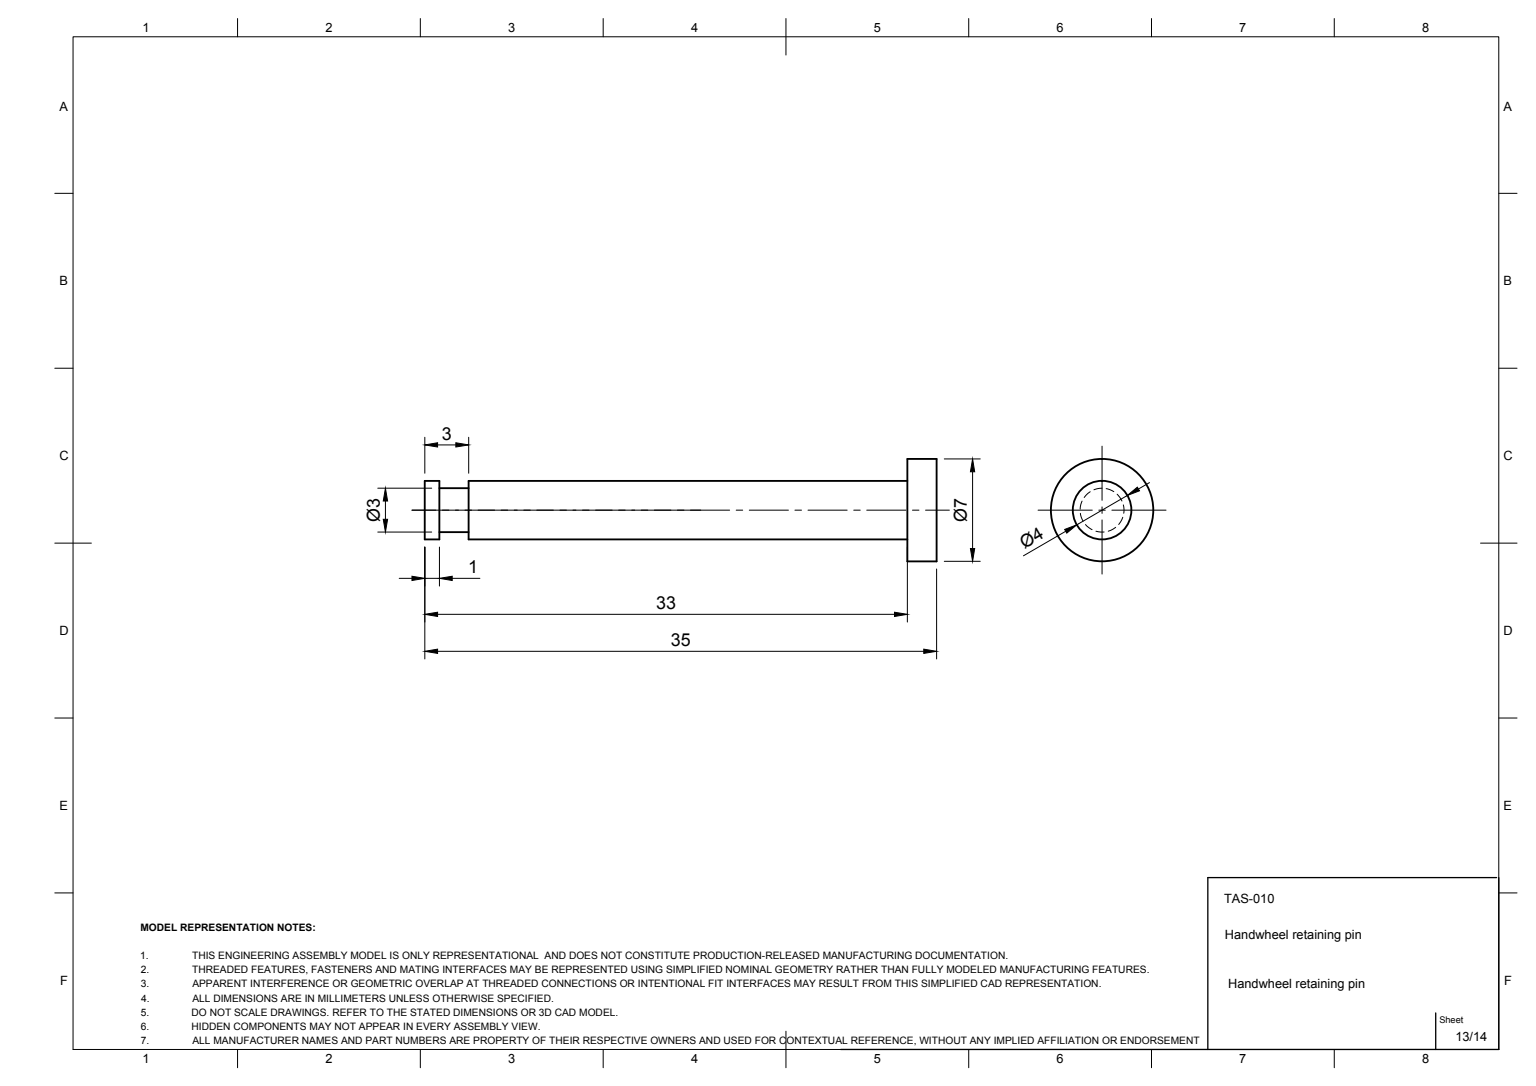
ISO-10303-21;
HEADER;
/* Generated by software containing ST-Developer
 * from STEP Tools, Inc. (www.steptools.com) 
 */

FILE_DESCRIPTION(
/* description */ (
'Independent keyed-quill tailstock, native coupled50mm slider andM16x2
 feed screw, conical dead center, bronze sleeves/thrust washers, cross
-pinned handwheel and bolted guide key. Custom center taper; no standa
rd taper compatibility, machine-bed compatibility or load rating assig
ned.'),
/* implementation_level */ '2;1');

FILE_NAME(
/* name */ 'Handwheel retaining pin.step',
/* time_stamp */ '2026-11-14T07:17:36-08:00',
/* author */ (''),
/* organization */ (''),
/* preprocessor_version */ 'ST-DEVELOPER v20.2',
/* originating_system */ 'Autodesk Translation Framework v15.17.0.0',
/* authorisation */ '');

FILE_SCHEMA (('AUTOMOTIVE_DESIGN { 1 0 10303 214 3 1 1 }'));
ENDSEC;

DATA;
#10=MECHANICAL_DESIGN_GEOMETRIC_PRESENTATION_REPRESENTATION('',(#163),#289387);
#129=SHAPE_REPRESENTATION_RELATIONSHIP('SRR','None',#289464,#146);
#146=ADVANCED_BREP_SHAPE_REPRESENTATION('',(#180),#289380);
#163=STYLED_ITEM('',(#289548),#180);
#180=MANIFOLD_SOLID_BREP('Body1',#16851);
#260=FACE_BOUND('',#1681,.T.);
#261=FACE_BOUND('',#1683,.T.);
#262=FACE_BOUND('',#1686,.T.);
#380=PLANE('',#17704);
#381=PLANE('',#17706);
#382=PLANE('',#17710);
#383=PLANE('',#17715);
#384=PLANE('',#17717);
#956=FACE_OUTER_BOUND('',#1679,.T.);
#957=FACE_OUTER_BOUND('',#1680,.T.);
#958=FACE_OUTER_BOUND('',#1682,.T.);
#959=FACE_OUTER_BOUND('',#1684,.T.);
#960=FACE_OUTER_BOUND('',#1685,.T.);
#961=FACE_OUTER_BOUND('',#1687,.T.);
#962=FACE_OUTER_BOUND('',#1688,.T.);
#963=FACE_OUTER_BOUND('',#1689,.T.);
#964=FACE_OUTER_BOUND('',#1690,.T.);
#1679=EDGE_LOOP('',(#14773,#14774,#14775,#14776));
#1680=EDGE_LOOP('',(#14777));
#1681=EDGE_LOOP('',(#14778));
#1682=EDGE_LOOP('',(#14779));
#1683=EDGE_LOOP('',(#14780));
#1684=EDGE_LOOP('',(#14781,#14782,#14783,#14784));
#1685=EDGE_LOOP('',(#14785));
#1686=EDGE_LOOP('',(#14786));
#1687=EDGE_LOOP('',(#14787,#14788,#14789,#14790));
#1688=EDGE_LOOP('',(#14791));
#1689=EDGE_LOOP('',(#14792,#14793,#14794,#14795));
#1690=EDGE_LOOP('',(#14796));
#1943=CIRCLE('',#17702,1.5);
#1944=CIRCLE('',#17703,1.5);
#1945=CIRCLE('',#17705,2.);
#1946=CIRCLE('',#17707,2.);
#1947=CIRCLE('',#17709,2.);
#1948=CIRCLE('',#17711,3.5);
#1949=CIRCLE('',#17712,2.);
#1950=CIRCLE('',#17714,3.5);
#4456=LINE('',#247266,#5093);
#4457=LINE('',#247277,#5094);
#4458=LINE('',#247285,#5095);
#4459=LINE('',#247289,#5096);
#5093=VECTOR('',#19718,1.5);
#5094=VECTOR('',#19733,2.);
#5095=VECTOR('',#19742,3.5);
#5096=VECTOR('',#19749,2.);
#7023=VERTEX_POINT('',#247263);
#7024=VERTEX_POINT('',#247265);
#7025=VERTEX_POINT('',#247269);
#7026=VERTEX_POINT('',#247272);
#7027=VERTEX_POINT('',#247275);
#7028=VERTEX_POINT('',#247279);
#7029=VERTEX_POINT('',#247281);
#7030=VERTEX_POINT('',#247284);
#9698=EDGE_CURVE('',#7023,#7023,#1943,.T.);
#9699=EDGE_CURVE('',#7023,#7024,#4456,.T.);
#9700=EDGE_CURVE('',#7024,#7024,#1944,.T.);
#9701=EDGE_CURVE('',#7025,#7025,#1945,.T.);
#9702=EDGE_CURVE('',#7026,#7026,#1946,.T.);
#9703=EDGE_CURVE('',#7027,#7027,#1947,.T.);
#9704=EDGE_CURVE('',#7027,#7026,#4457,.T.);
#9705=EDGE_CURVE('',#7028,#7028,#1948,.T.);
#9706=EDGE_CURVE('',#7029,#7029,#1949,.T.);
#9707=EDGE_CURVE('',#7028,#7030,#4458,.T.);
#9708=EDGE_CURVE('',#7030,#7030,#1950,.T.);
#9709=EDGE_CURVE('',#7025,#7029,#4459,.T.);
#14773=ORIENTED_EDGE('',*,*,#9698,.F.);
#14774=ORIENTED_EDGE('',*,*,#9699,.T.);
#14775=ORIENTED_EDGE('',*,*,#9700,.T.);
#14776=ORIENTED_EDGE('',*,*,#9699,.F.);
#14777=ORIENTED_EDGE('',*,*,#9701,.F.);
#14778=ORIENTED_EDGE('',*,*,#9700,.F.);
#14779=ORIENTED_EDGE('',*,*,#9702,.F.);
#14780=ORIENTED_EDGE('',*,*,#9698,.T.);
#14781=ORIENTED_EDGE('',*,*,#9703,.F.);
#14782=ORIENTED_EDGE('',*,*,#9704,.T.);
#14783=ORIENTED_EDGE('',*,*,#9702,.T.);
#14784=ORIENTED_EDGE('',*,*,#9704,.F.);
#14785=ORIENTED_EDGE('',*,*,#9705,.T.);
#14786=ORIENTED_EDGE('',*,*,#9706,.F.);
#14787=ORIENTED_EDGE('',*,*,#9705,.F.);
#14788=ORIENTED_EDGE('',*,*,#9707,.T.);
#14789=ORIENTED_EDGE('',*,*,#9708,.T.);
#14790=ORIENTED_EDGE('',*,*,#9707,.F.);
#14791=ORIENTED_EDGE('',*,*,#9708,.F.);
#14792=ORIENTED_EDGE('',*,*,#9701,.T.);
#14793=ORIENTED_EDGE('',*,*,#9709,.T.);
#14794=ORIENTED_EDGE('',*,*,#9706,.T.);
#14795=ORIENTED_EDGE('',*,*,#9709,.F.);
#14796=ORIENTED_EDGE('',*,*,#9703,.T.);
#16128=CYLINDRICAL_SURFACE('',#17701,1.5);
#16129=CYLINDRICAL_SURFACE('',#17708,2.);
#16130=CYLINDRICAL_SURFACE('',#17713,3.5);
#16131=CYLINDRICAL_SURFACE('',#17716,2.);
#16724=ADVANCED_FACE('',(#956),#16128,.T.);
#16725=ADVANCED_FACE('',(#957,#260),#380,.F.);
#16726=ADVANCED_FACE('',(#958,#261),#381,.F.);
#16727=ADVANCED_FACE('',(#959),#16129,.T.);
#16728=ADVANCED_FACE('',(#960,#262),#382,.T.);
#16729=ADVANCED_FACE('',(#961),#16130,.T.);
#16730=ADVANCED_FACE('',(#962),#383,.F.);
#16731=ADVANCED_FACE('',(#963),#16131,.T.);
#16732=ADVANCED_FACE('',(#964),#384,.T.);
#16851=CLOSED_SHELL('',(#16724,#16725,#16726,#16727,#16728,#16729,#16730,
#16731,#16732));
#17700=AXIS2_PLACEMENT_3D('',#247261,#19712,#19713);
#17701=AXIS2_PLACEMENT_3D('',#247262,#19714,#19715);
#17702=AXIS2_PLACEMENT_3D('',#247264,#19716,#19717);
#17703=AXIS2_PLACEMENT_3D('',#247267,#19719,#19720);
#17704=AXIS2_PLACEMENT_3D('',#247268,#19721,#19722);
#17705=AXIS2_PLACEMENT_3D('',#247270,#19723,#19724);
#17706=AXIS2_PLACEMENT_3D('',#247271,#19725,#19726);
#17707=AXIS2_PLACEMENT_3D('',#247273,#19727,#19728);
#17708=AXIS2_PLACEMENT_3D('',#247274,#19729,#19730);
#17709=AXIS2_PLACEMENT_3D('',#247276,#19731,#19732);
#17710=AXIS2_PLACEMENT_3D('',#247278,#19734,#19735);
#17711=AXIS2_PLACEMENT_3D('',#247280,#19736,#19737);
#17712=AXIS2_PLACEMENT_3D('',#247282,#19738,#19739);
#17713=AXIS2_PLACEMENT_3D('',#247283,#19740,#19741);
#17714=AXIS2_PLACEMENT_3D('',#247286,#19743,#19744);
#17715=AXIS2_PLACEMENT_3D('',#247287,#19745,#19746);
#17716=AXIS2_PLACEMENT_3D('',#247288,#19747,#19748);
#17717=AXIS2_PLACEMENT_3D('',#247290,#19750,#19751);
#19712=DIRECTION('axis',(0.,0.,1.));
#19713=DIRECTION('refdir',(1.,0.,0.));
#19714=DIRECTION('center_axis',(0.,0.,1.));
#19715=DIRECTION('ref_axis',(1.,0.,0.));
#19716=DIRECTION('center_axis',(0.,0.,1.));
#19717=DIRECTION('ref_axis',(1.,0.,0.));
#19718=DIRECTION('',(0.,0.,-1.));
#19719=DIRECTION('center_axis',(0.,0.,1.));
#19720=DIRECTION('ref_axis',(1.,0.,0.));
#19721=DIRECTION('center_axis',(0.,0.,-1.));
#19722=DIRECTION('ref_axis',(-1.,0.,0.));
#19723=DIRECTION('center_axis',(0.,0.,-1.));
#19724=DIRECTION('ref_axis',(1.,0.,0.));
#19725=DIRECTION('center_axis',(0.,0.,1.));
#19726=DIRECTION('ref_axis',(1.,0.,0.));
#19727=DIRECTION('center_axis',(0.,0.,1.));
#19728=DIRECTION('ref_axis',(1.,0.,0.));
#19729=DIRECTION('center_axis',(0.,0.,1.));
#19730=DIRECTION('ref_axis',(1.,0.,0.));
#19731=DIRECTION('center_axis',(0.,0.,1.));
#19732=DIRECTION('ref_axis',(1.,0.,0.));
#19733=DIRECTION('',(0.,0.,-1.));
#19734=DIRECTION('center_axis',(0.,0.,1.));
#19735=DIRECTION('ref_axis',(1.,0.,0.));
#19736=DIRECTION('center_axis',(0.,0.,1.));
#19737=DIRECTION('ref_axis',(1.,0.,0.));
#19738=DIRECTION('center_axis',(0.,0.,1.));
#19739=DIRECTION('ref_axis',(1.,0.,0.));
#19740=DIRECTION('center_axis',(0.,0.,1.));
#19741=DIRECTION('ref_axis',(1.,0.,0.));
#19742=DIRECTION('',(0.,0.,-1.));
#19743=DIRECTION('center_axis',(0.,0.,1.));
#19744=DIRECTION('ref_axis',(1.,0.,0.));
#19745=DIRECTION('center_axis',(0.,0.,1.));
#19746=DIRECTION('ref_axis',(1.,0.,0.));
#19747=DIRECTION('center_axis',(0.,0.,1.));
#19748=DIRECTION('ref_axis',(1.,0.,0.));
#19749=DIRECTION('',(0.,0.,-1.));
#19750=DIRECTION('center_axis',(0.,0.,1.));
#19751=DIRECTION('ref_axis',(1.,0.,0.));
#247261=CARTESIAN_POINT('',(0.,0.,0.));
#247262=CARTESIAN_POINT('Origin',(0.,0.,31.));
#247263=CARTESIAN_POINT('',(-1.5,-1.83697019872103E-16,32.));
#247264=CARTESIAN_POINT('Origin',(0.,0.,32.));
#247265=CARTESIAN_POINT('',(-1.5,-1.83697019872103E-16,30.));
#247266=CARTESIAN_POINT('',(-1.5,-1.83697019872103E-16,31.));
#247267=CARTESIAN_POINT('Origin',(0.,0.,30.));
#247268=CARTESIAN_POINT('Origin',(5.5,0.,30.));
#247269=CARTESIAN_POINT('',(-2.,2.44929359829471E-16,30.));
#247270=CARTESIAN_POINT('Origin',(0.,0.,30.));
#247271=CARTESIAN_POINT('Origin',(1.5,0.,32.));
#247272=CARTESIAN_POINT('',(-2.,-2.44929359829471E-16,32.));
#247273=CARTESIAN_POINT('Origin',(0.,0.,32.));
#247274=CARTESIAN_POINT('Origin',(0.,0.,0.));
#247275=CARTESIAN_POINT('',(-2.,-2.44929359829471E-16,33.));
#247276=CARTESIAN_POINT('Origin',(0.,0.,33.));
#247277=CARTESIAN_POINT('',(-2.,-2.44929359829471E-16,0.));
#247278=CARTESIAN_POINT('Origin',(0.,0.,0.));
#247279=CARTESIAN_POINT('',(-3.5,-4.28626379701574E-16,0.));
#247280=CARTESIAN_POINT('Origin',(0.,0.,0.));
#247281=CARTESIAN_POINT('',(-2.,-2.44929359829471E-16,0.));
#247282=CARTESIAN_POINT('Origin',(0.,0.,0.));
#247283=CARTESIAN_POINT('Origin',(0.,0.,-2.));
#247284=CARTESIAN_POINT('',(-3.5,-4.28626379701574E-16,-2.));
#247285=CARTESIAN_POINT('',(-3.5,-4.28626379701574E-16,-2.));
#247286=CARTESIAN_POINT('Origin',(0.,0.,-2.));
#247287=CARTESIAN_POINT('Origin',(0.,0.,-2.));
#247288=CARTESIAN_POINT('Origin',(0.,0.,0.));
#247289=CARTESIAN_POINT('',(-2.,-2.44929359829471E-16,0.));
#247290=CARTESIAN_POINT('Origin',(0.,0.,33.));
#289361=UNCERTAINTY_MEASURE_WITH_UNIT(LENGTH_MEASURE(0.01),#289388,
'DISTANCE_ACCURACY_VALUE',
'Maximum model space distance between geometric entities at asserted c
onnectivities');
#289368=UNCERTAINTY_MEASURE_WITH_UNIT(LENGTH_MEASURE(0.01),#289388,
'DISTANCE_ACCURACY_VALUE',
'Maximum model space distance between geometric entities at asserted c
onnectivities');
#289380=(
GEOMETRIC_REPRESENTATION_CONTEXT(3)
GLOBAL_UNCERTAINTY_ASSIGNED_CONTEXT((#289361))
GLOBAL_UNIT_ASSIGNED_CONTEXT((#289388,#289390,#289391))
REPRESENTATION_CONTEXT('','3D')
);
#289387=(
GEOMETRIC_REPRESENTATION_CONTEXT(3)
GLOBAL_UNCERTAINTY_ASSIGNED_CONTEXT((#289368))
GLOBAL_UNIT_ASSIGNED_CONTEXT((#289388,#289390,#289391))
REPRESENTATION_CONTEXT('','3D')
);
#289388=(
LENGTH_UNIT()
NAMED_UNIT(*)
SI_UNIT(.MILLI.,.METRE.)
);
#289390=(
NAMED_UNIT(*)
PLANE_ANGLE_UNIT()
SI_UNIT($,.RADIAN.)
);
#289391=(
NAMED_UNIT(*)
SI_UNIT($,.STERADIAN.)
SOLID_ANGLE_UNIT()
);
#289403=SHAPE_DEFINITION_REPRESENTATION(#289421,#289464);
#289421=PRODUCT_DEFINITION_SHAPE('',$,#289483);
#289464=SHAPE_REPRESENTATION('',(#17700),#289380);
#289471=PRODUCT_DEFINITION_CONTEXT('part definition',#289527,'design');
#289483=PRODUCT_DEFINITION('Handwheel retaining pin',
'Handwheel retaining pin',#289501,#289471);
#289501=PRODUCT_DEFINITION_FORMATION('',$,#289540);
#289527=APPLICATION_CONTEXT(
'Core Data for Automotive Mechanical Design Process');
#289528=PRODUCT_CONTEXT('part definition',#289527,'mechanical');
#289540=PRODUCT('Handwheel retaining pin','Handwheel retaining pin',$,(#289528));
#289548=PRESENTATION_STYLE_ASSIGNMENT((#289555));
#289555=SURFACE_STYLE_USAGE(.BOTH.,#289562);
#289562=SURFACE_SIDE_STYLE('',(#289569));
#289569=SURFACE_STYLE_FILL_AREA(#289576);
#289576=FILL_AREA_STYLE('Opaque(104,114,127)',(#289583));
#289583=FILL_AREA_STYLE_COLOUR('Opaque(104,114,127)',#289590);
#289590=COLOUR_RGB('Opaque(104,114,127)',0.407843137254902,0.447058823529412,
0.498039215686275);
ENDSEC;
END-ISO-10303-21;
